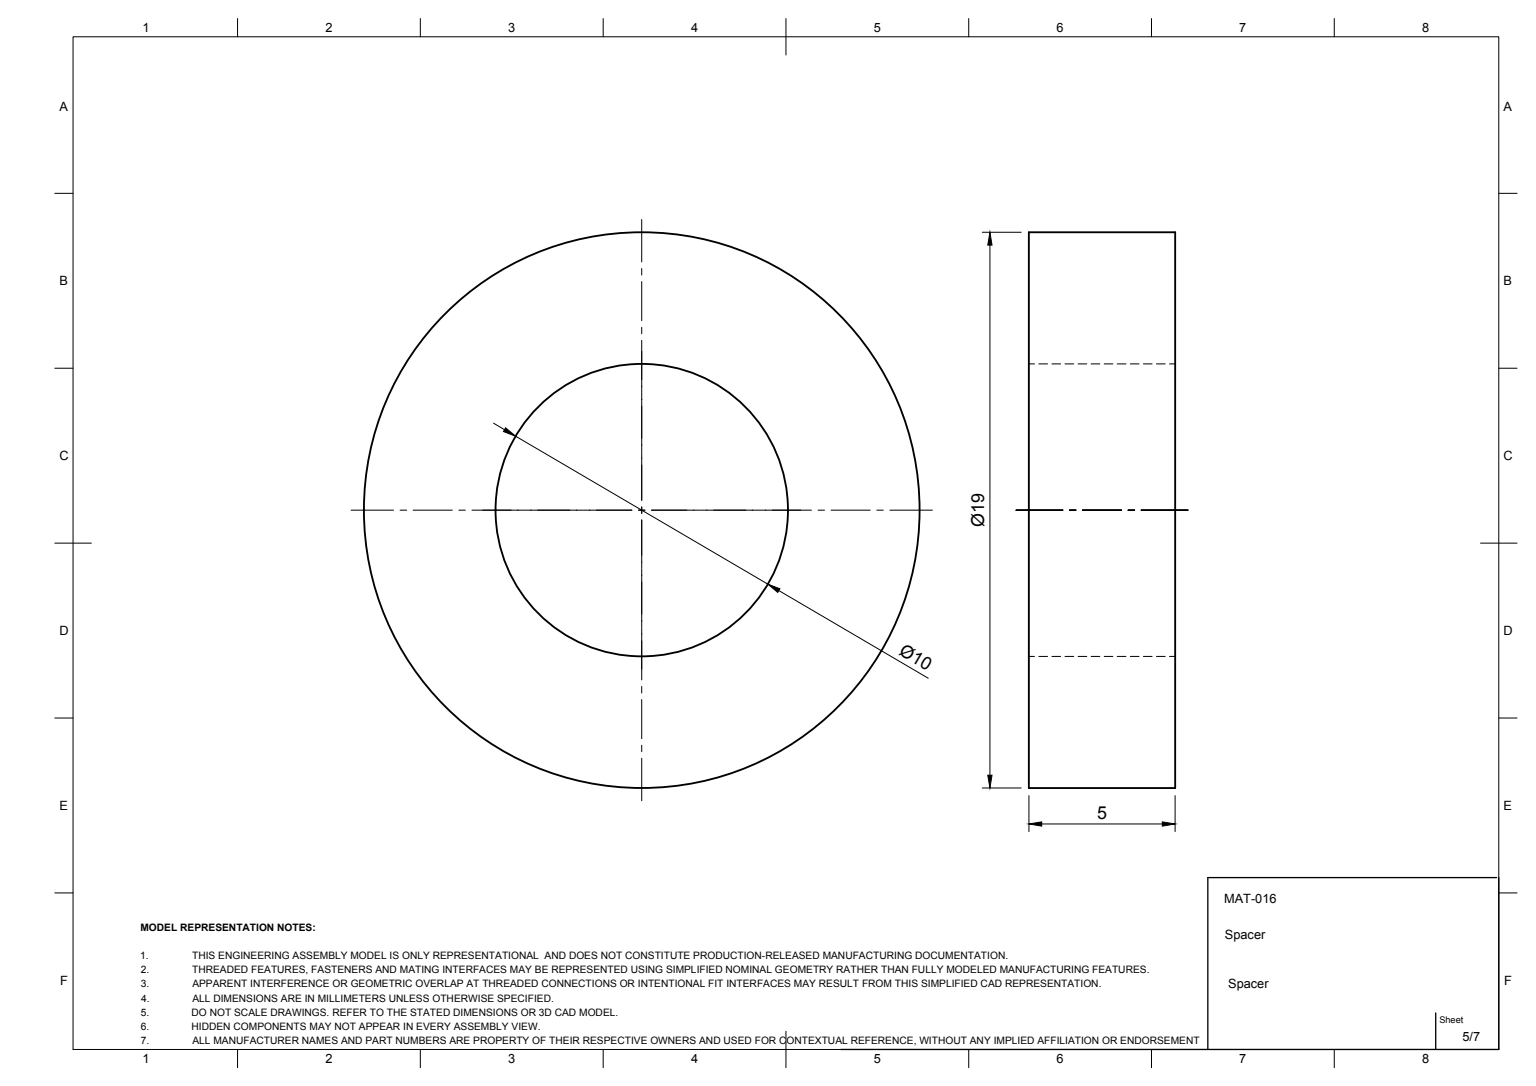
ISO-10303-21;
HEADER;
/* Generated by software containing ST-Developer
 * from STEP Tools, Inc. (www.steptools.com) 
 */

FILE_DESCRIPTION(
/* description */ ('STEP AP214'),
/* implementation_level */ '2;1');

FILE_NAME(
/* name */ 'Spacer.step',
/* time_stamp */ '2026-11-14T06:10:26-08:00',
/* author */ (''),
/* organization */ (''),
/* preprocessor_version */ 'ST-DEVELOPER v20.2',
/* originating_system */ 'Autodesk Translation Framework v15.17.0.0',
/* authorisation */ '');

FILE_SCHEMA (('AUTOMOTIVE_DESIGN { 1 0 10303 214 3 1 1 }'));
ENDSEC;

DATA;
#10=MECHANICAL_DESIGN_GEOMETRIC_PRESENTATION_REPRESENTATION('',(#169),#10413);
#153=SHAPE_REPRESENTATION_RELATIONSHIP('SRR','None',#10458,#161);
#161=ADVANCED_BREP_SHAPE_REPRESENTATION('',(#177),#10410);
#169=STYLED_ITEM('',(#10503),#177);
#177=MANIFOLD_SOLID_BREP('Body1',#5304);
#214=FACE_BOUND('',#854,.T.);
#215=FACE_BOUND('',#856,.T.);
#256=PLANE('',#6083);
#257=PLANE('',#6084);
#527=FACE_OUTER_BOUND('',#851,.T.);
#528=FACE_OUTER_BOUND('',#852,.T.);
#529=FACE_OUTER_BOUND('',#853,.T.);
#530=FACE_OUTER_BOUND('',#855,.T.);
#851=EDGE_LOOP('',(#4610,#4611,#4612,#4613));
#852=EDGE_LOOP('',(#4614,#4615,#4616,#4617));
#853=EDGE_LOOP('',(#4618));
#854=EDGE_LOOP('',(#4619));
#855=EDGE_LOOP('',(#4620));
#856=EDGE_LOOP('',(#4621));
#1142=LINE('',#9412,#1433);
#1143=LINE('',#9418,#1434);
#1433=VECTOR('',#7764,5.);
#1434=VECTOR('',#7771,9.5);
#1898=CIRCLE('',#6078,5.);
#1899=CIRCLE('',#6079,5.);
#1900=CIRCLE('',#6081,9.5);
#1901=CIRCLE('',#6082,9.5);
#2375=VERTEX_POINT('',#9409);
#2376=VERTEX_POINT('',#9411);
#2377=VERTEX_POINT('',#9415);
#2378=VERTEX_POINT('',#9417);
#3130=EDGE_CURVE('',#2375,#2375,#1898,.T.);
#3131=EDGE_CURVE('',#2375,#2376,#1142,.T.);
#3132=EDGE_CURVE('',#2376,#2376,#1899,.T.);
#3133=EDGE_CURVE('',#2377,#2377,#1900,.T.);
#3134=EDGE_CURVE('',#2377,#2378,#1143,.T.);
#3135=EDGE_CURVE('',#2378,#2378,#1901,.T.);
#4610=ORIENTED_EDGE('',*,*,#3130,.T.);
#4611=ORIENTED_EDGE('',*,*,#3131,.T.);
#4612=ORIENTED_EDGE('',*,*,#3132,.F.);
#4613=ORIENTED_EDGE('',*,*,#3131,.F.);
#4614=ORIENTED_EDGE('',*,*,#3133,.T.);
#4615=ORIENTED_EDGE('',*,*,#3134,.T.);
#4616=ORIENTED_EDGE('',*,*,#3135,.F.);
#4617=ORIENTED_EDGE('',*,*,#3134,.F.);
#4618=ORIENTED_EDGE('',*,*,#3135,.T.);
#4619=ORIENTED_EDGE('',*,*,#3130,.F.);
#4620=ORIENTED_EDGE('',*,*,#3133,.F.);
#4621=ORIENTED_EDGE('',*,*,#3132,.T.);
#4997=CYLINDRICAL_SURFACE('',#6077,5.);
#4998=CYLINDRICAL_SURFACE('',#6080,9.5);
#5261=ADVANCED_FACE('',(#527),#4997,.F.);
#5262=ADVANCED_FACE('',(#528),#4998,.T.);
#5263=ADVANCED_FACE('',(#529,#214),#256,.T.);
#5264=ADVANCED_FACE('',(#530,#215),#257,.F.);
#5304=CLOSED_SHELL('',(#5261,#5262,#5263,#5264));
#6076=AXIS2_PLACEMENT_3D('',#9407,#7758,#7759);
#6077=AXIS2_PLACEMENT_3D('',#9408,#7760,#7761);
#6078=AXIS2_PLACEMENT_3D('',#9410,#7762,#7763);
#6079=AXIS2_PLACEMENT_3D('',#9413,#7765,#7766);
#6080=AXIS2_PLACEMENT_3D('',#9414,#7767,#7768);
#6081=AXIS2_PLACEMENT_3D('',#9416,#7769,#7770);
#6082=AXIS2_PLACEMENT_3D('',#9419,#7772,#7773);
#6083=AXIS2_PLACEMENT_3D('',#9420,#7774,#7775);
#6084=AXIS2_PLACEMENT_3D('',#9421,#7776,#7777);
#7758=DIRECTION('axis',(0.,0.,1.));
#7759=DIRECTION('refdir',(1.,0.,0.));
#7760=DIRECTION('center_axis',(0.,0.,-1.));
#7761=DIRECTION('ref_axis',(-1.,0.,0.));
#7762=DIRECTION('center_axis',(0.,0.,1.));
#7763=DIRECTION('ref_axis',(1.,0.,0.));
#7764=DIRECTION('',(0.,0.,-1.));
#7765=DIRECTION('center_axis',(0.,0.,1.));
#7766=DIRECTION('ref_axis',(1.,0.,0.));
#7767=DIRECTION('center_axis',(0.,0.,-1.));
#7768=DIRECTION('ref_axis',(-1.,0.,0.));
#7769=DIRECTION('center_axis',(0.,0.,1.));
#7770=DIRECTION('ref_axis',(1.,0.,0.));
#7771=DIRECTION('',(0.,0.,1.));
#7772=DIRECTION('center_axis',(0.,0.,1.));
#7773=DIRECTION('ref_axis',(1.,0.,0.));
#7774=DIRECTION('center_axis',(0.,0.,1.));
#7775=DIRECTION('ref_axis',(1.,0.,0.));
#7776=DIRECTION('center_axis',(0.,0.,1.));
#7777=DIRECTION('ref_axis',(1.,0.,0.));
#9407=CARTESIAN_POINT('',(0.,0.,0.));
#9408=CARTESIAN_POINT('Origin',(0.,0.,5.));
#9409=CARTESIAN_POINT('',(5.,-6.12323399573677E-16,5.));
#9410=CARTESIAN_POINT('Origin',(0.,0.,5.));
#9411=CARTESIAN_POINT('',(5.,-6.12323399573677E-16,0.));
#9412=CARTESIAN_POINT('',(5.,-6.12323399573677E-16,5.));
#9413=CARTESIAN_POINT('Origin',(0.,0.,0.));
#9414=CARTESIAN_POINT('Origin',(0.,0.,5.));
#9415=CARTESIAN_POINT('',(9.5,-1.16341445918999E-15,5.55111512312578E-16));
#9416=CARTESIAN_POINT('Origin',(0.,0.,0.));
#9417=CARTESIAN_POINT('',(9.5,-1.16341445918999E-15,5.));
#9418=CARTESIAN_POINT('',(9.5,-1.16341445918999E-15,5.));
#9419=CARTESIAN_POINT('Origin',(0.,0.,5.));
#9420=CARTESIAN_POINT('Origin',(0.,0.,5.));
#9421=CARTESIAN_POINT('Origin',(0.,0.,0.));
#10400=UNCERTAINTY_MEASURE_WITH_UNIT(LENGTH_MEASURE(0.01),#10414,
'DISTANCE_ACCURACY_VALUE',
'Maximum model space distance between geometric entities at asserted c
onnectivities');
#10403=UNCERTAINTY_MEASURE_WITH_UNIT(LENGTH_MEASURE(0.01),#10414,
'DISTANCE_ACCURACY_VALUE',
'Maximum model space distance between geometric entities at asserted c
onnectivities');
#10410=(
GEOMETRIC_REPRESENTATION_CONTEXT(3)
GLOBAL_UNCERTAINTY_ASSIGNED_CONTEXT((#10400))
GLOBAL_UNIT_ASSIGNED_CONTEXT((#10414,#10416,#10417))
REPRESENTATION_CONTEXT('','3D')
);
#10413=(
GEOMETRIC_REPRESENTATION_CONTEXT(3)
GLOBAL_UNCERTAINTY_ASSIGNED_CONTEXT((#10403))
GLOBAL_UNIT_ASSIGNED_CONTEXT((#10414,#10416,#10417))
REPRESENTATION_CONTEXT('','3D')
);
#10414=(
LENGTH_UNIT()
NAMED_UNIT(*)
SI_UNIT(.MILLI.,.METRE.)
);
#10416=(
NAMED_UNIT(*)
PLANE_ANGLE_UNIT()
SI_UNIT($,.RADIAN.)
);
#10417=(
NAMED_UNIT(*)
SI_UNIT($,.STERADIAN.)
SOLID_ANGLE_UNIT()
);
#10424=SHAPE_DEFINITION_REPRESENTATION(#10433,#10458);
#10433=PRODUCT_DEFINITION_SHAPE('',$,#10468);
#10458=SHAPE_REPRESENTATION('',(#6076),#10410);
#10461=PRODUCT_DEFINITION_CONTEXT('part definition',#10490,'design');
#10468=PRODUCT_DEFINITION('Spacer','Spacer',#10477,#10461);
#10477=PRODUCT_DEFINITION_FORMATION('',$,#10498);
#10490=APPLICATION_CONTEXT(
'Core Data for Automotive Mechanical Design Process');
#10491=PRODUCT_CONTEXT('part definition',#10490,'mechanical');
#10498=PRODUCT('Spacer','Spacer',$,(#10491));
#10503=PRESENTATION_STYLE_ASSIGNMENT((#10507));
#10507=SURFACE_STYLE_USAGE(.BOTH.,#10511);
#10511=SURFACE_SIDE_STYLE('',(#10515));
#10515=SURFACE_STYLE_FILL_AREA(#10519);
#10519=FILL_AREA_STYLE('Opaque(97,158,199)',(#10523));
#10523=FILL_AREA_STYLE_COLOUR('Opaque(97,158,199)',#10527);
#10527=COLOUR_RGB('Opaque(97,158,199)',0.380392156862745,0.619607843137255,
0.780392156862745);
ENDSEC;
END-ISO-10303-21;
